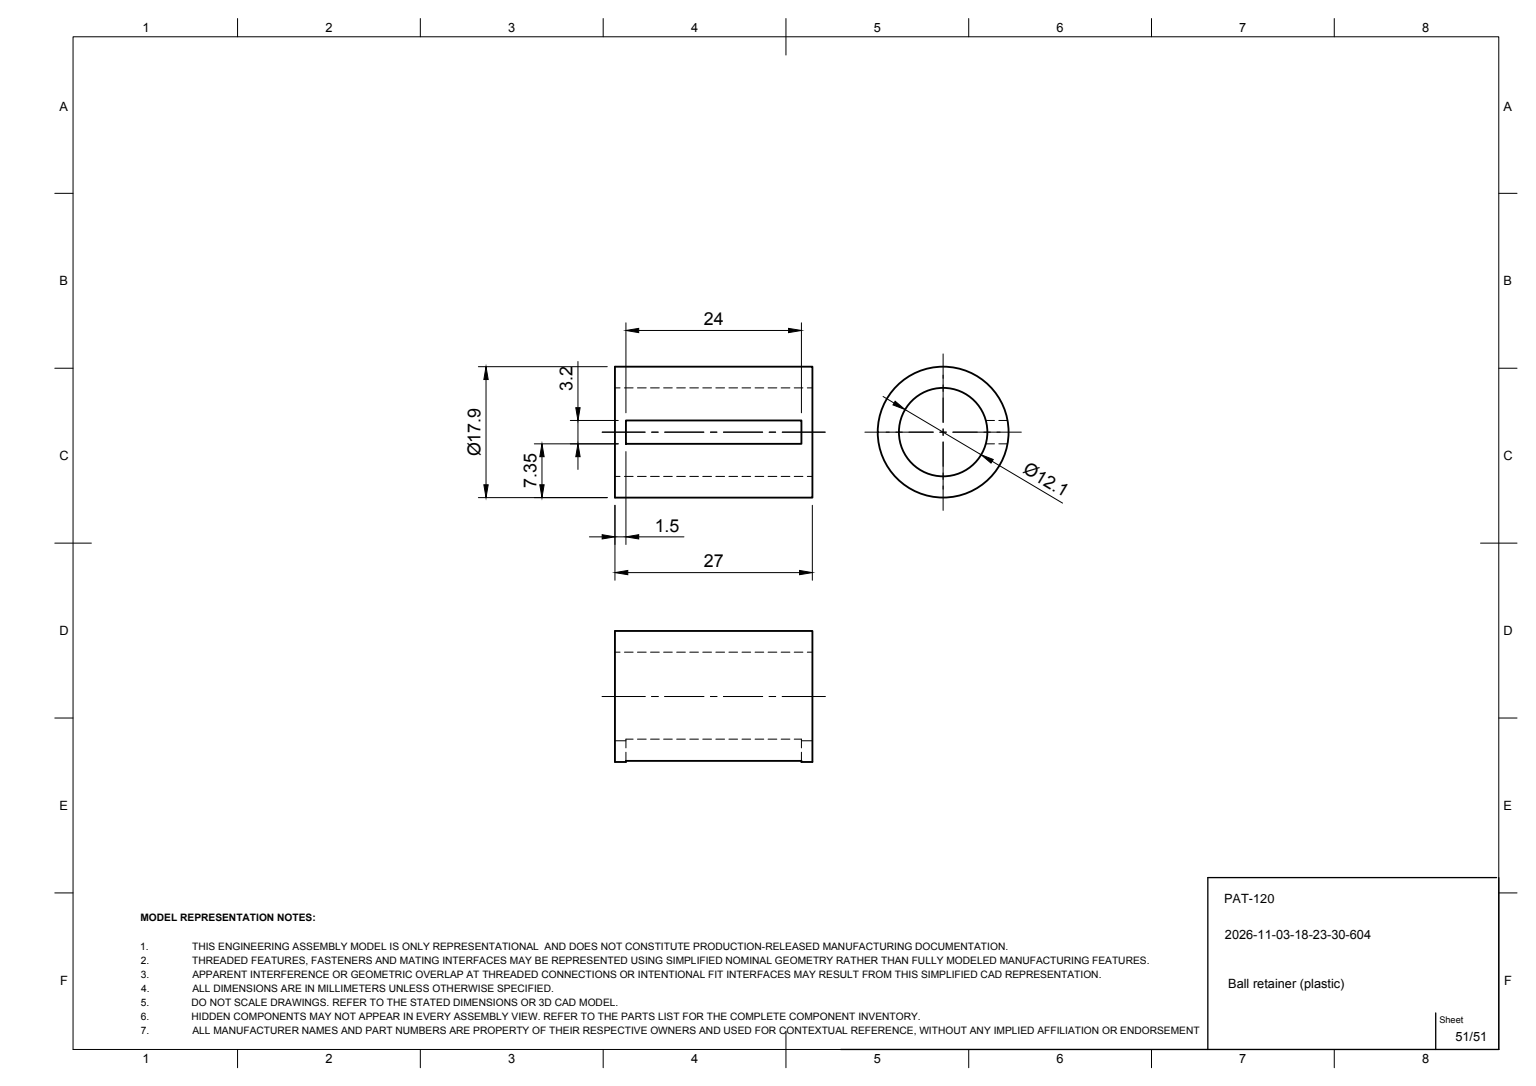
ISO-10303-21;
HEADER;
/* Generated by software containing ST-Developer
 * from STEP Tools, Inc. (www.steptools.com) 
 */

FILE_DESCRIPTION(
/* description */ ('Vibration shaker table dummy'),
/* implementation_level */ '2;1');

FILE_NAME(
/* name */ 'Ball retainer (plastic).step',
/* time_stamp */ '2026-10-27T10:55:14-07:00',
/* author */ (''),
/* organization */ (''),
/* preprocessor_version */ 'ST-DEVELOPER v20.2',
/* originating_system */ 'Autodesk Translation Framework v15.17.0.0',
/* authorisation */ '');

FILE_SCHEMA (('AUTOMOTIVE_DESIGN { 1 0 10303 214 3 1 1 }'));
ENDSEC;

DATA;
#10=MECHANICAL_DESIGN_GEOMETRIC_PRESENTATION_REPRESENTATION('',(#730),#22394);
#638=SHAPE_REPRESENTATION_RELATIONSHIP('SRR','None',#22686,#684);
#684=ADVANCED_BREP_SHAPE_REPRESENTATION('',(#774),#22392);
#730=STYLED_ITEM('',(#22954),#774);
#774=MANIFOLD_SOLID_BREP('Body1',#9250);
#1055=FACE_BOUND('',#2597,.T.);
#1056=FACE_BOUND('',#2599,.T.);
#1057=FACE_BOUND('',#2601,.T.);
#1058=FACE_BOUND('',#2603,.T.);
#1324=PLANE('',#10769);
#1325=PLANE('',#10772);
#1326=PLANE('',#10773);
#1327=PLANE('',#10776);
#1328=PLANE('',#10777);
#1329=PLANE('',#10782);
#1814=FACE_OUTER_BOUND('',#2592,.T.);
#1815=FACE_OUTER_BOUND('',#2593,.T.);
#1816=FACE_OUTER_BOUND('',#2594,.T.);
#1817=FACE_OUTER_BOUND('',#2595,.T.);
#1818=FACE_OUTER_BOUND('',#2596,.T.);
#1819=FACE_OUTER_BOUND('',#2598,.T.);
#1820=FACE_OUTER_BOUND('',#2600,.T.);
#1821=FACE_OUTER_BOUND('',#2602,.T.);
#2592=EDGE_LOOP('',(#8406,#8407,#8408,#8409));
#2593=EDGE_LOOP('',(#8410,#8411,#8412,#8413));
#2594=EDGE_LOOP('',(#8414,#8415,#8416,#8417));
#2595=EDGE_LOOP('',(#8418,#8419,#8420,#8421));
#2596=EDGE_LOOP('',(#8422));
#2597=EDGE_LOOP('',(#8423));
#2598=EDGE_LOOP('',(#8424,#8425,#8426,#8427));
#2599=EDGE_LOOP('',(#8428,#8429,#8430,#8431));
#2600=EDGE_LOOP('',(#8432));
#2601=EDGE_LOOP('',(#8433));
#2602=EDGE_LOOP('',(#8434,#8435,#8436,#8437));
#2603=EDGE_LOOP('',(#8438,#8439,#8440,#8441));
#3207=LINE('',#22051,#3826);
#3208=LINE('',#22054,#3827);
#3209=LINE('',#22057,#3828);
#3210=LINE('',#22059,#3829);
#3211=LINE('',#22060,#3830);
#3212=LINE('',#22066,#3831);
#3213=LINE('',#22068,#3832);
#3214=LINE('',#22069,#3833);
#3215=LINE('',#22078,#3834);
#3216=LINE('',#22083,#3835);
#3826=VECTOR('',#13557,1.);
#3827=VECTOR('',#13560,1.);
#3828=VECTOR('',#13563,1.);
#3829=VECTOR('',#13564,1.);
#3830=VECTOR('',#13565,1.);
#3831=VECTOR('',#13572,1.);
#3832=VECTOR('',#13575,1.);
#3833=VECTOR('',#13576,1.);
#3834=VECTOR('',#13587,0.895);
#3835=VECTOR('',#13594,0.605);
#4351=CIRCLE('',#10770,0.895);
#4352=CIRCLE('',#10771,0.605);
#4353=CIRCLE('',#10774,0.895);
#4354=CIRCLE('',#10775,0.605);
#4355=CIRCLE('',#10778,0.895);
#4356=CIRCLE('',#10779,0.605);
#4357=CIRCLE('',#10781,0.895);
#4358=CIRCLE('',#10783,0.605);
#5084=VERTEX_POINT('',#22047);
#5085=VERTEX_POINT('',#22048);
#5086=VERTEX_POINT('',#22050);
#5087=VERTEX_POINT('',#22052);
#5088=VERTEX_POINT('',#22056);
#5089=VERTEX_POINT('',#22058);
#5090=VERTEX_POINT('',#22062);
#5091=VERTEX_POINT('',#22064);
#5092=VERTEX_POINT('',#22071);
#5093=VERTEX_POINT('',#22073);
#5094=VERTEX_POINT('',#22076);
#5095=VERTEX_POINT('',#22080);
#6196=EDGE_CURVE('',#5084,#5085,#4351,.T.);
#6197=EDGE_CURVE('',#5086,#5084,#3207,.T.);
#6198=EDGE_CURVE('',#5087,#5086,#4352,.T.);
#6199=EDGE_CURVE('',#5085,#5087,#3208,.T.);
#6200=EDGE_CURVE('',#5085,#5088,#3209,.T.);
#6201=EDGE_CURVE('',#5089,#5087,#3210,.T.);
#6202=EDGE_CURVE('',#5089,#5088,#3211,.T.);
#6203=EDGE_CURVE('',#5088,#5090,#4353,.T.);
#6204=EDGE_CURVE('',#5091,#5089,#4354,.T.);
#6205=EDGE_CURVE('',#5090,#5091,#3212,.T.);
#6206=EDGE_CURVE('',#5090,#5084,#3213,.T.);
#6207=EDGE_CURVE('',#5086,#5091,#3214,.T.);
#6208=EDGE_CURVE('',#5092,#5092,#4355,.T.);
#6209=EDGE_CURVE('',#5093,#5093,#4356,.T.);
#6210=EDGE_CURVE('',#5094,#5094,#4357,.T.);
#6211=EDGE_CURVE('',#5094,#5092,#3215,.T.);
#6212=EDGE_CURVE('',#5095,#5095,#4358,.T.);
#6213=EDGE_CURVE('',#5095,#5093,#3216,.T.);
#8406=ORIENTED_EDGE('',*,*,#6196,.F.);
#8407=ORIENTED_EDGE('',*,*,#6197,.F.);
#8408=ORIENTED_EDGE('',*,*,#6198,.F.);
#8409=ORIENTED_EDGE('',*,*,#6199,.F.);
#8410=ORIENTED_EDGE('',*,*,#6200,.F.);
#8411=ORIENTED_EDGE('',*,*,#6199,.T.);
#8412=ORIENTED_EDGE('',*,*,#6201,.F.);
#8413=ORIENTED_EDGE('',*,*,#6202,.T.);
#8414=ORIENTED_EDGE('',*,*,#6203,.F.);
#8415=ORIENTED_EDGE('',*,*,#6202,.F.);
#8416=ORIENTED_EDGE('',*,*,#6204,.F.);
#8417=ORIENTED_EDGE('',*,*,#6205,.F.);
#8418=ORIENTED_EDGE('',*,*,#6206,.F.);
#8419=ORIENTED_EDGE('',*,*,#6205,.T.);
#8420=ORIENTED_EDGE('',*,*,#6207,.F.);
#8421=ORIENTED_EDGE('',*,*,#6197,.T.);
#8422=ORIENTED_EDGE('',*,*,#6208,.F.);
#8423=ORIENTED_EDGE('',*,*,#6209,.T.);
#8424=ORIENTED_EDGE('',*,*,#6210,.F.);
#8425=ORIENTED_EDGE('',*,*,#6211,.T.);
#8426=ORIENTED_EDGE('',*,*,#6208,.T.);
#8427=ORIENTED_EDGE('',*,*,#6211,.F.);
#8428=ORIENTED_EDGE('',*,*,#6203,.T.);
#8429=ORIENTED_EDGE('',*,*,#6206,.T.);
#8430=ORIENTED_EDGE('',*,*,#6196,.T.);
#8431=ORIENTED_EDGE('',*,*,#6200,.T.);
#8432=ORIENTED_EDGE('',*,*,#6210,.T.);
#8433=ORIENTED_EDGE('',*,*,#6212,.F.);
#8434=ORIENTED_EDGE('',*,*,#6212,.T.);
#8435=ORIENTED_EDGE('',*,*,#6213,.T.);
#8436=ORIENTED_EDGE('',*,*,#6209,.F.);
#8437=ORIENTED_EDGE('',*,*,#6213,.F.);
#8438=ORIENTED_EDGE('',*,*,#6204,.T.);
#8439=ORIENTED_EDGE('',*,*,#6201,.T.);
#8440=ORIENTED_EDGE('',*,*,#6198,.T.);
#8441=ORIENTED_EDGE('',*,*,#6207,.T.);
#8702=CYLINDRICAL_SURFACE('',#10780,0.895);
#8703=CYLINDRICAL_SURFACE('',#10784,0.605);
#9179=ADVANCED_FACE('',(#1814),#1324,.F.);
#9180=ADVANCED_FACE('',(#1815),#1325,.F.);
#9181=ADVANCED_FACE('',(#1816),#1326,.F.);
#9182=ADVANCED_FACE('',(#1817),#1327,.F.);
#9183=ADVANCED_FACE('',(#1818,#1055),#1328,.T.);
#9184=ADVANCED_FACE('',(#1819,#1056),#8702,.T.);
#9185=ADVANCED_FACE('',(#1820,#1057),#1329,.T.);
#9186=ADVANCED_FACE('',(#1821,#1058),#8703,.F.);
#9250=CLOSED_SHELL('',(#9179,#9180,#9181,#9182,#9183,#9184,#9185,#9186));
#10768=AXIS2_PLACEMENT_3D('',#22045,#13551,#13552);
#10769=AXIS2_PLACEMENT_3D('',#22046,#13553,#13554);
#10770=AXIS2_PLACEMENT_3D('',#22049,#13555,#13556);
#10771=AXIS2_PLACEMENT_3D('',#22053,#13558,#13559);
#10772=AXIS2_PLACEMENT_3D('',#22055,#13561,#13562);
#10773=AXIS2_PLACEMENT_3D('',#22061,#13566,#13567);
#10774=AXIS2_PLACEMENT_3D('',#22063,#13568,#13569);
#10775=AXIS2_PLACEMENT_3D('',#22065,#13570,#13571);
#10776=AXIS2_PLACEMENT_3D('',#22067,#13573,#13574);
#10777=AXIS2_PLACEMENT_3D('',#22070,#13577,#13578);
#10778=AXIS2_PLACEMENT_3D('',#22072,#13579,#13580);
#10779=AXIS2_PLACEMENT_3D('',#22074,#13581,#13582);
#10780=AXIS2_PLACEMENT_3D('',#22075,#13583,#13584);
#10781=AXIS2_PLACEMENT_3D('',#22077,#13585,#13586);
#10782=AXIS2_PLACEMENT_3D('',#22079,#13588,#13589);
#10783=AXIS2_PLACEMENT_3D('',#22081,#13590,#13591);
#10784=AXIS2_PLACEMENT_3D('',#22082,#13592,#13593);
#13551=DIRECTION('axis',(0.,0.,1.));
#13552=DIRECTION('refdir',(1.,0.,0.));
#13553=DIRECTION('center_axis',(0.,1.,0.));
#13554=DIRECTION('ref_axis',(0.,0.,1.));
#13555=DIRECTION('center_axis',(0.,1.,0.));
#13556=DIRECTION('ref_axis',(1.,0.,0.));
#13557=DIRECTION('',(1.,0.,0.));
#13558=DIRECTION('center_axis',(0.,-1.,0.));
#13559=DIRECTION('ref_axis',(1.,0.,0.));
#13560=DIRECTION('',(-1.,0.,0.));
#13561=DIRECTION('center_axis',(0.,0.,-1.));
#13562=DIRECTION('ref_axis',(-1.,0.,0.));
#13563=DIRECTION('',(0.,-1.,0.));
#13564=DIRECTION('',(0.,1.,0.));
#13565=DIRECTION('',(1.,0.,0.));
#13566=DIRECTION('center_axis',(0.,-1.,0.));
#13567=DIRECTION('ref_axis',(0.,0.,-1.));
#13568=DIRECTION('center_axis',(0.,-1.,0.));
#13569=DIRECTION('ref_axis',(1.,0.,0.));
#13570=DIRECTION('center_axis',(0.,1.,0.));
#13571=DIRECTION('ref_axis',(1.,0.,0.));
#13572=DIRECTION('',(-1.,0.,0.));
#13573=DIRECTION('center_axis',(0.,0.,1.));
#13574=DIRECTION('ref_axis',(1.,0.,0.));
#13575=DIRECTION('',(0.,1.,0.));
#13576=DIRECTION('',(0.,-1.,0.));
#13577=DIRECTION('center_axis',(0.,1.,0.));
#13578=DIRECTION('ref_axis',(0.,0.,1.));
#13579=DIRECTION('center_axis',(0.,-1.,0.));
#13580=DIRECTION('ref_axis',(1.,0.,0.));
#13581=DIRECTION('center_axis',(0.,-1.,0.));
#13582=DIRECTION('ref_axis',(1.,0.,0.));
#13583=DIRECTION('center_axis',(0.,-1.,0.));
#13584=DIRECTION('ref_axis',(1.,0.,0.));
#13585=DIRECTION('center_axis',(0.,-1.,0.));
#13586=DIRECTION('ref_axis',(1.,0.,0.));
#13587=DIRECTION('',(0.,1.,0.));
#13588=DIRECTION('center_axis',(0.,-1.,0.));
#13589=DIRECTION('ref_axis',(0.,0.,-1.));
#13590=DIRECTION('center_axis',(0.,-1.,0.));
#13591=DIRECTION('ref_axis',(1.,0.,0.));
#13592=DIRECTION('center_axis',(0.,-1.,0.));
#13593=DIRECTION('ref_axis',(1.,0.,0.));
#13594=DIRECTION('',(0.,1.,0.));
#22045=CARTESIAN_POINT('',(0.,0.,0.));
#22046=CARTESIAN_POINT('Origin',(0.75,1.2,0.));
#22047=CARTESIAN_POINT('',(0.880582193778639,1.2,0.16));
#22048=CARTESIAN_POINT('',(0.880582193778639,1.2,-0.16));
#22049=CARTESIAN_POINT('Origin',(0.,1.2,0.));
#22050=CARTESIAN_POINT('',(0.583459510163302,1.2,0.16));
#22051=CARTESIAN_POINT('',(0.57,1.2,0.16));
#22052=CARTESIAN_POINT('',(0.583459510163302,1.2,-0.16));
#22053=CARTESIAN_POINT('Origin',(0.,1.2,0.));
#22054=CARTESIAN_POINT('',(0.93,1.2,-0.16));
#22055=CARTESIAN_POINT('Origin',(0.93,0.,-0.16));
#22056=CARTESIAN_POINT('',(0.880582193778639,-1.2,-0.16));
#22057=CARTESIAN_POINT('',(0.880582193778639,0.,-0.16));
#22058=CARTESIAN_POINT('',(0.583459510163302,-1.2,-0.16));
#22059=CARTESIAN_POINT('',(0.583459510163302,0.,-0.16));
#22060=CARTESIAN_POINT('',(0.93,-1.2,-0.16));
#22061=CARTESIAN_POINT('Origin',(0.75,-1.2,0.));
#22062=CARTESIAN_POINT('',(0.880582193778639,-1.2,0.16));
#22063=CARTESIAN_POINT('Origin',(0.,-1.2,0.));
#22064=CARTESIAN_POINT('',(0.583459510163302,-1.2,0.16));
#22065=CARTESIAN_POINT('Origin',(0.,-1.2,0.));
#22066=CARTESIAN_POINT('',(0.57,-1.2,0.16));
#22067=CARTESIAN_POINT('Origin',(0.57,0.,0.16));
#22068=CARTESIAN_POINT('',(0.880582193778639,0.,0.16));
#22069=CARTESIAN_POINT('',(0.583459510163302,0.,0.16));
#22070=CARTESIAN_POINT('Origin',(0.895,1.35,0.));
#22071=CARTESIAN_POINT('',(-0.895,1.35,-1.09605888523688E-16));
#22072=CARTESIAN_POINT('Origin',(0.,1.35,0.));
#22073=CARTESIAN_POINT('',(-0.605,1.35,-7.40911313484149E-17));
#22074=CARTESIAN_POINT('Origin',(0.,1.35,0.));
#22075=CARTESIAN_POINT('Origin',(0.,0.,0.));
#22076=CARTESIAN_POINT('',(-0.895,-1.35,-1.09605888523688E-16));
#22077=CARTESIAN_POINT('Origin',(0.,-1.35,0.));
#22078=CARTESIAN_POINT('',(-0.895,0.,-1.09605888523688E-16));
#22079=CARTESIAN_POINT('Origin',(0.605,-1.35,0.));
#22080=CARTESIAN_POINT('',(-0.605,-1.35,-7.40911313484149E-17));
#22081=CARTESIAN_POINT('Origin',(0.,-1.35,0.));
#22082=CARTESIAN_POINT('Origin',(0.,0.,0.));
#22083=CARTESIAN_POINT('',(-0.605,0.,-7.40911313484149E-17));
#22341=UNCERTAINTY_MEASURE_WITH_UNIT(LENGTH_MEASURE(0.001),#22395,
'DISTANCE_ACCURACY_VALUE',
'Maximum model space distance between geometric entities at asserted c
onnectivities');
#22343=UNCERTAINTY_MEASURE_WITH_UNIT(LENGTH_MEASURE(0.001),#22395,
'DISTANCE_ACCURACY_VALUE',
'Maximum model space distance between geometric entities at asserted c
onnectivities');
#22392=(
GEOMETRIC_REPRESENTATION_CONTEXT(3)
GLOBAL_UNCERTAINTY_ASSIGNED_CONTEXT((#22341))
GLOBAL_UNIT_ASSIGNED_CONTEXT((#22395,#22397,#22398))
REPRESENTATION_CONTEXT('','3D')
);
#22394=(
GEOMETRIC_REPRESENTATION_CONTEXT(3)
GLOBAL_UNCERTAINTY_ASSIGNED_CONTEXT((#22343))
GLOBAL_UNIT_ASSIGNED_CONTEXT((#22395,#22397,#22398))
REPRESENTATION_CONTEXT('','3D')
);
#22395=(
LENGTH_UNIT()
NAMED_UNIT(*)
SI_UNIT(.CENTI.,.METRE.)
);
#22397=(
NAMED_UNIT(*)
PLANE_ANGLE_UNIT()
SI_UNIT($,.RADIAN.)
);
#22398=(
NAMED_UNIT(*)
SI_UNIT($,.STERADIAN.)
SOLID_ANGLE_UNIT()
);
#22447=SHAPE_DEFINITION_REPRESENTATION(#22497,#22686);
#22497=PRODUCT_DEFINITION_SHAPE('',$,#22737);
#22686=SHAPE_REPRESENTATION('',(#10768),#22392);
#22688=PRODUCT_DEFINITION_CONTEXT('part definition',#22840,'design');
#22737=PRODUCT_DEFINITION('Ball retainer (plastic)',
'Ball retainer (plastic)',#22787,#22688);
#22787=PRODUCT_DEFINITION_FORMATION('',$,#22890);
#22840=APPLICATION_CONTEXT(
'Core Data for Automotive Mechanical Design Process');
#22841=PRODUCT_CONTEXT('part definition',#22840,'mechanical');
#22890=PRODUCT('Ball retainer (plastic)','Ball retainer (plastic)',
'Ball retainer (plastic)',(#22841));
#22948=COLOUR_RGB('Sky Blue',0.24,0.69,0.87);
#22949=FILL_AREA_STYLE_COLOUR('',#22948);
#22950=FILL_AREA_STYLE('',(#22949));
#22951=SURFACE_STYLE_FILL_AREA(#22950);
#22952=SURFACE_SIDE_STYLE('',(#22951));
#22953=SURFACE_STYLE_USAGE(.BOTH.,#22952);
#22954=PRESENTATION_STYLE_ASSIGNMENT((#22953));
ENDSEC;
END-ISO-10303-21;
